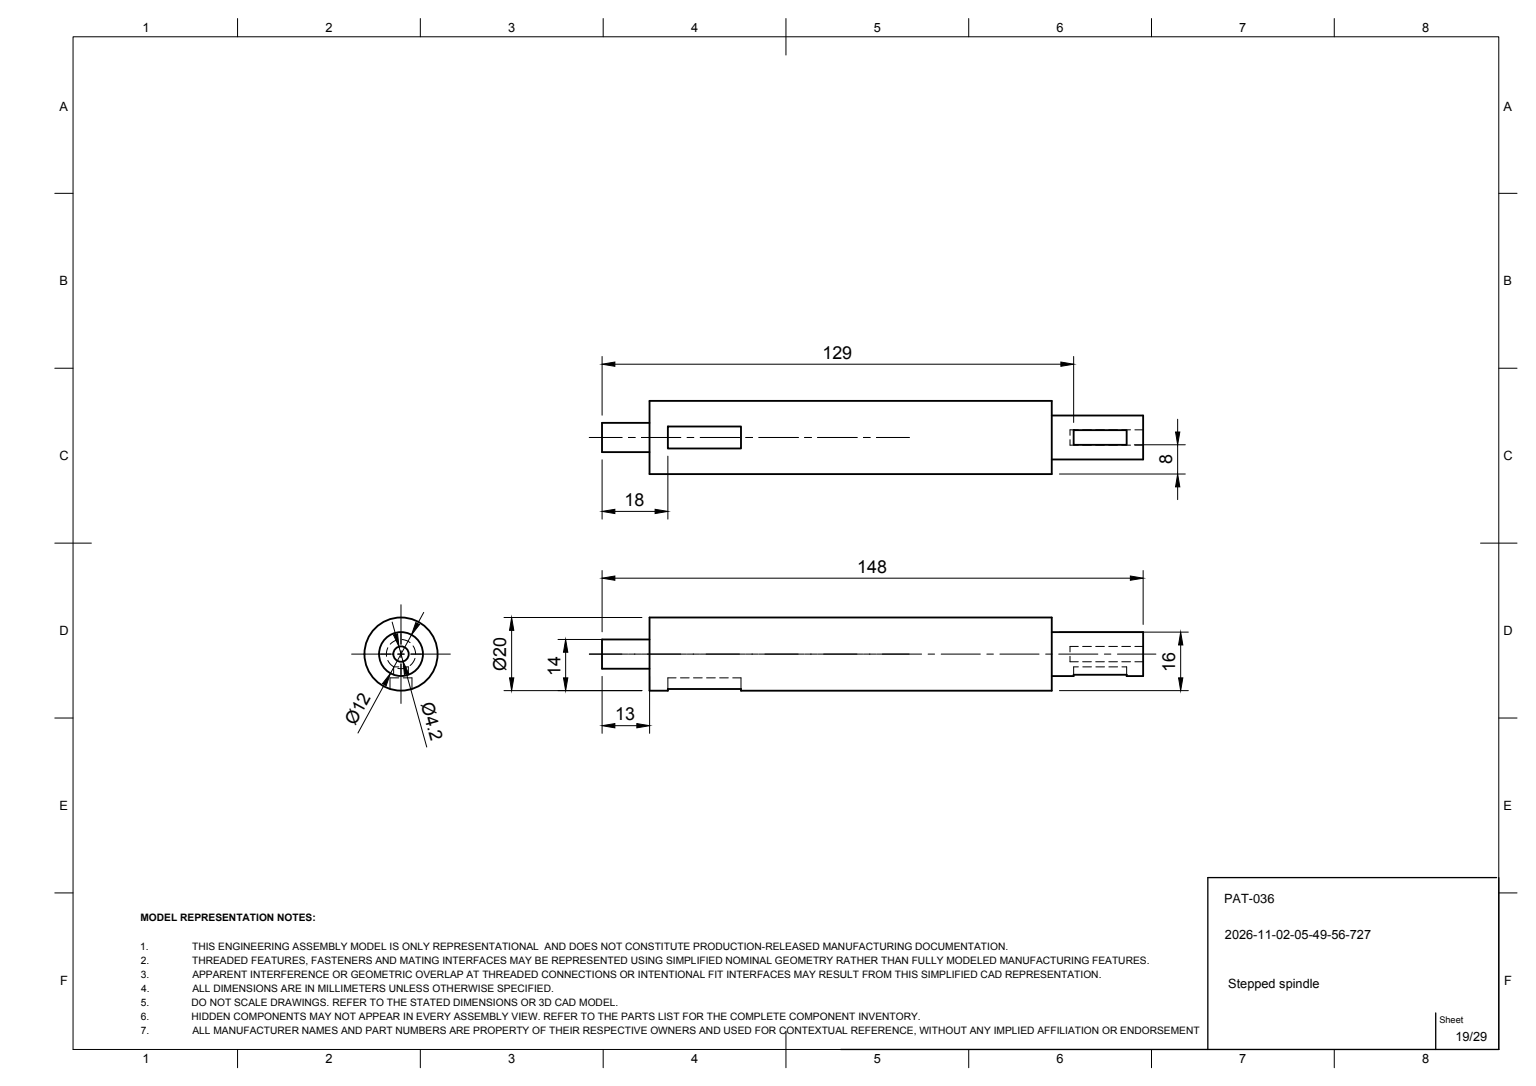
ISO-10303-21;
HEADER;
/* Generated by software containing ST-Developer
 * from STEP Tools, Inc. (www.steptools.com) 
 */

FILE_DESCRIPTION(
/* description */ ('Flange-mounted spindle'),
/* implementation_level */ '2;1');

FILE_NAME(
/* name */ 'Stepped spindle.step',
/* time_stamp */ '2026-10-27T10:49:51-07:00',
/* author */ (''),
/* organization */ (''),
/* preprocessor_version */ 'ST-DEVELOPER v20.2',
/* originating_system */ 'Autodesk Translation Framework v15.17.0.0',
/* authorisation */ '');

FILE_SCHEMA (('AUTOMOTIVE_DESIGN { 1 0 10303 214 3 1 1 }'));
ENDSEC;

DATA;
#10=MECHANICAL_DESIGN_GEOMETRIC_PRESENTATION_REPRESENTATION('',(#351),#11764);
#296=SHAPE_REPRESENTATION_RELATIONSHIP('SRR','None',#11894,#323);
#323=ADVANCED_BREP_SHAPE_REPRESENTATION('',(#377),#11749);
#351=STYLED_ITEM('',(#12085),#377);
#377=MANIFOLD_SOLID_BREP('Body1',#6145);
#452=FACE_BOUND('',#1216,.T.);
#453=FACE_BOUND('',#1218,.T.);
#454=FACE_BOUND('',#1220,.T.);
#455=FACE_BOUND('',#1222,.T.);
#456=FACE_BOUND('',#1224,.T.);
#579=PLANE('',#6676);
#580=PLANE('',#6677);
#581=PLANE('',#6679);
#582=PLANE('',#6680);
#583=PLANE('',#6681);
#584=PLANE('',#6686);
#585=PLANE('',#6687);
#586=PLANE('',#6688);
#587=PLANE('',#6690);
#588=PLANE('',#6691);
#589=PLANE('',#6692);
#590=PLANE('',#6697);
#591=PLANE('',#6701);
#592=PLANE('',#6705);
#593=PLANE('',#6706);
#795=FACE_OUTER_BOUND('',#1201,.T.);
#796=FACE_OUTER_BOUND('',#1202,.T.);
#797=FACE_OUTER_BOUND('',#1203,.T.);
#798=FACE_OUTER_BOUND('',#1204,.T.);
#799=FACE_OUTER_BOUND('',#1205,.T.);
#800=FACE_OUTER_BOUND('',#1206,.T.);
#801=FACE_OUTER_BOUND('',#1207,.T.);
#802=FACE_OUTER_BOUND('',#1208,.T.);
#803=FACE_OUTER_BOUND('',#1209,.T.);
#804=FACE_OUTER_BOUND('',#1210,.T.);
#805=FACE_OUTER_BOUND('',#1211,.T.);
#806=FACE_OUTER_BOUND('',#1212,.T.);
#807=FACE_OUTER_BOUND('',#1213,.T.);
#808=FACE_OUTER_BOUND('',#1214,.T.);
#809=FACE_OUTER_BOUND('',#1215,.T.);
#810=FACE_OUTER_BOUND('',#1217,.T.);
#811=FACE_OUTER_BOUND('',#1219,.T.);
#812=FACE_OUTER_BOUND('',#1221,.T.);
#813=FACE_OUTER_BOUND('',#1223,.T.);
#1201=EDGE_LOOP('',(#4527,#4528,#4529,#4530));
#1202=EDGE_LOOP('',(#4531,#4532,#4533,#4534));
#1203=EDGE_LOOP('',(#4535,#4536,#4537,#4538));
#1204=EDGE_LOOP('',(#4539,#4540,#4541,#4542));
#1205=EDGE_LOOP('',(#4543,#4544,#4545,#4546));
#1206=EDGE_LOOP('',(#4547,#4548,#4549,#4550));
#1207=EDGE_LOOP('',(#4551));
#1208=EDGE_LOOP('',(#4552,#4553,#4554,#4555));
#1209=EDGE_LOOP('',(#4556,#4557,#4558,#4559));
#1210=EDGE_LOOP('',(#4560,#4561,#4562,#4563));
#1211=EDGE_LOOP('',(#4564,#4565,#4566,#4567));
#1212=EDGE_LOOP('',(#4568,#4569,#4570,#4571));
#1213=EDGE_LOOP('',(#4572,#4573,#4574,#4575));
#1214=EDGE_LOOP('',(#4576));
#1215=EDGE_LOOP('',(#4577,#4578,#4579,#4580));
#1216=EDGE_LOOP('',(#4581,#4582,#4583,#4584));
#1217=EDGE_LOOP('',(#4585));
#1218=EDGE_LOOP('',(#4586));
#1219=EDGE_LOOP('',(#4587,#4588,#4589,#4590));
#1220=EDGE_LOOP('',(#4591,#4592,#4593,#4594));
#1221=EDGE_LOOP('',(#4595));
#1222=EDGE_LOOP('',(#4596));
#1223=EDGE_LOOP('',(#4597));
#1224=EDGE_LOOP('',(#4598));
#1639=LINE('',#10119,#2061);
#1640=LINE('',#10121,#2062);
#1641=LINE('',#10123,#2063);
#1642=LINE('',#10124,#2064);
#1643=LINE('',#10129,#2065);
#1644=LINE('',#10130,#2066);
#1645=LINE('',#10133,#2067);
#1646=LINE('',#10135,#2068);
#1647=LINE('',#10136,#2069);
#1648=LINE('',#10138,#2070);
#1649=LINE('',#10145,#2071);
#1650=LINE('',#10151,#2072);
#1651=LINE('',#10153,#2073);
#1652=LINE('',#10155,#2074);
#1653=LINE('',#10156,#2075);
#1654=LINE('',#10161,#2076);
#1655=LINE('',#10162,#2077);
#1656=LINE('',#10165,#2078);
#1657=LINE('',#10167,#2079);
#1658=LINE('',#10168,#2080);
#1659=LINE('',#10170,#2081);
#1660=LINE('',#10177,#2082);
#1661=LINE('',#10184,#2083);
#1662=LINE('',#10191,#2084);
#2061=VECTOR('',#7804,1.);
#2062=VECTOR('',#7805,1.);
#2063=VECTOR('',#7806,1.);
#2064=VECTOR('',#7807,1.);
#2065=VECTOR('',#7812,1.);
#2066=VECTOR('',#7813,1.);
#2067=VECTOR('',#7816,1.);
#2068=VECTOR('',#7817,1.);
#2069=VECTOR('',#7818,1.);
#2070=VECTOR('',#7821,1.);
#2071=VECTOR('',#7830,0.21);
#2072=VECTOR('',#7837,1.);
#2073=VECTOR('',#7838,1.);
#2074=VECTOR('',#7839,1.);
#2075=VECTOR('',#7840,1.);
#2076=VECTOR('',#7845,1.);
#2077=VECTOR('',#7846,1.);
#2078=VECTOR('',#7849,1.);
#2079=VECTOR('',#7850,1.);
#2080=VECTOR('',#7851,1.);
#2081=VECTOR('',#7854,1.);
#2082=VECTOR('',#7863,0.4);
#2083=VECTOR('',#7872,0.6);
#2084=VECTOR('',#7881,1.);
#2400=CIRCLE('',#6678,1.);
#2401=CIRCLE('',#6682,1.);
#2402=CIRCLE('',#6684,0.21);
#2403=CIRCLE('',#6685,0.21);
#2404=CIRCLE('',#6689,0.6);
#2405=CIRCLE('',#6693,0.6);
#2406=CIRCLE('',#6695,0.4);
#2407=CIRCLE('',#6696,0.4);
#2408=CIRCLE('',#6699,0.6);
#2409=CIRCLE('',#6700,0.6);
#2410=CIRCLE('',#6703,1.);
#2411=CIRCLE('',#6704,1.);
#2828=VERTEX_POINT('',#10117);
#2829=VERTEX_POINT('',#10118);
#2830=VERTEX_POINT('',#10120);
#2831=VERTEX_POINT('',#10122);
#2832=VERTEX_POINT('',#10126);
#2833=VERTEX_POINT('',#10128);
#2834=VERTEX_POINT('',#10132);
#2835=VERTEX_POINT('',#10134);
#2836=VERTEX_POINT('',#10142);
#2837=VERTEX_POINT('',#10144);
#2838=VERTEX_POINT('',#10149);
#2839=VERTEX_POINT('',#10150);
#2840=VERTEX_POINT('',#10152);
#2841=VERTEX_POINT('',#10154);
#2842=VERTEX_POINT('',#10158);
#2843=VERTEX_POINT('',#10160);
#2844=VERTEX_POINT('',#10164);
#2845=VERTEX_POINT('',#10166);
#2846=VERTEX_POINT('',#10174);
#2847=VERTEX_POINT('',#10176);
#2848=VERTEX_POINT('',#10181);
#2849=VERTEX_POINT('',#10183);
#2850=VERTEX_POINT('',#10188);
#2851=VERTEX_POINT('',#10190);
#3456=EDGE_CURVE('',#2828,#2829,#1639,.T.);
#3457=EDGE_CURVE('',#2828,#2830,#1640,.T.);
#3458=EDGE_CURVE('',#2831,#2830,#1641,.T.);
#3459=EDGE_CURVE('',#2831,#2829,#1642,.T.);
#3460=EDGE_CURVE('',#2829,#2832,#2400,.T.);
#3461=EDGE_CURVE('',#2833,#2831,#1643,.T.);
#3462=EDGE_CURVE('',#2832,#2833,#1644,.T.);
#3463=EDGE_CURVE('',#2832,#2834,#1645,.T.);
#3464=EDGE_CURVE('',#2833,#2835,#1646,.T.);
#3465=EDGE_CURVE('',#2835,#2834,#1647,.T.);
#3466=EDGE_CURVE('',#2830,#2835,#1648,.T.);
#3467=EDGE_CURVE('',#2834,#2828,#2401,.T.);
#3468=EDGE_CURVE('',#2836,#2836,#2402,.T.);
#3469=EDGE_CURVE('',#2836,#2837,#1649,.T.);
#3470=EDGE_CURVE('',#2837,#2837,#2403,.T.);
#3471=EDGE_CURVE('',#2838,#2839,#1650,.T.);
#3472=EDGE_CURVE('',#2838,#2840,#1651,.T.);
#3473=EDGE_CURVE('',#2841,#2840,#1652,.T.);
#3474=EDGE_CURVE('',#2841,#2839,#1653,.T.);
#3475=EDGE_CURVE('',#2839,#2842,#2404,.T.);
#3476=EDGE_CURVE('',#2843,#2841,#1654,.T.);
#3477=EDGE_CURVE('',#2842,#2843,#1655,.T.);
#3478=EDGE_CURVE('',#2842,#2844,#1656,.T.);
#3479=EDGE_CURVE('',#2843,#2845,#1657,.T.);
#3480=EDGE_CURVE('',#2845,#2844,#1658,.T.);
#3481=EDGE_CURVE('',#2840,#2845,#1659,.T.);
#3482=EDGE_CURVE('',#2844,#2838,#2405,.T.);
#3483=EDGE_CURVE('',#2846,#2846,#2406,.T.);
#3484=EDGE_CURVE('',#2846,#2847,#1660,.T.);
#3485=EDGE_CURVE('',#2847,#2847,#2407,.T.);
#3486=EDGE_CURVE('',#2848,#2848,#2408,.T.);
#3487=EDGE_CURVE('',#2848,#2849,#1661,.T.);
#3488=EDGE_CURVE('',#2849,#2849,#2409,.T.);
#3489=EDGE_CURVE('',#2850,#2850,#2410,.T.);
#3490=EDGE_CURVE('',#2850,#2851,#1662,.T.);
#3491=EDGE_CURVE('',#2851,#2851,#2411,.T.);
#4527=ORIENTED_EDGE('',*,*,#3456,.F.);
#4528=ORIENTED_EDGE('',*,*,#3457,.T.);
#4529=ORIENTED_EDGE('',*,*,#3458,.F.);
#4530=ORIENTED_EDGE('',*,*,#3459,.T.);
#4531=ORIENTED_EDGE('',*,*,#3460,.F.);
#4532=ORIENTED_EDGE('',*,*,#3459,.F.);
#4533=ORIENTED_EDGE('',*,*,#3461,.F.);
#4534=ORIENTED_EDGE('',*,*,#3462,.F.);
#4535=ORIENTED_EDGE('',*,*,#3463,.F.);
#4536=ORIENTED_EDGE('',*,*,#3462,.T.);
#4537=ORIENTED_EDGE('',*,*,#3464,.T.);
#4538=ORIENTED_EDGE('',*,*,#3465,.T.);
#4539=ORIENTED_EDGE('',*,*,#3461,.T.);
#4540=ORIENTED_EDGE('',*,*,#3458,.T.);
#4541=ORIENTED_EDGE('',*,*,#3466,.T.);
#4542=ORIENTED_EDGE('',*,*,#3464,.F.);
#4543=ORIENTED_EDGE('',*,*,#3467,.F.);
#4544=ORIENTED_EDGE('',*,*,#3465,.F.);
#4545=ORIENTED_EDGE('',*,*,#3466,.F.);
#4546=ORIENTED_EDGE('',*,*,#3457,.F.);
#4547=ORIENTED_EDGE('',*,*,#3468,.F.);
#4548=ORIENTED_EDGE('',*,*,#3469,.T.);
#4549=ORIENTED_EDGE('',*,*,#3470,.T.);
#4550=ORIENTED_EDGE('',*,*,#3469,.F.);
#4551=ORIENTED_EDGE('',*,*,#3470,.F.);
#4552=ORIENTED_EDGE('',*,*,#3471,.F.);
#4553=ORIENTED_EDGE('',*,*,#3472,.T.);
#4554=ORIENTED_EDGE('',*,*,#3473,.F.);
#4555=ORIENTED_EDGE('',*,*,#3474,.T.);
#4556=ORIENTED_EDGE('',*,*,#3475,.F.);
#4557=ORIENTED_EDGE('',*,*,#3474,.F.);
#4558=ORIENTED_EDGE('',*,*,#3476,.F.);
#4559=ORIENTED_EDGE('',*,*,#3477,.F.);
#4560=ORIENTED_EDGE('',*,*,#3478,.F.);
#4561=ORIENTED_EDGE('',*,*,#3477,.T.);
#4562=ORIENTED_EDGE('',*,*,#3479,.T.);
#4563=ORIENTED_EDGE('',*,*,#3480,.T.);
#4564=ORIENTED_EDGE('',*,*,#3476,.T.);
#4565=ORIENTED_EDGE('',*,*,#3473,.T.);
#4566=ORIENTED_EDGE('',*,*,#3481,.T.);
#4567=ORIENTED_EDGE('',*,*,#3479,.F.);
#4568=ORIENTED_EDGE('',*,*,#3482,.F.);
#4569=ORIENTED_EDGE('',*,*,#3480,.F.);
#4570=ORIENTED_EDGE('',*,*,#3481,.F.);
#4571=ORIENTED_EDGE('',*,*,#3472,.F.);
#4572=ORIENTED_EDGE('',*,*,#3483,.F.);
#4573=ORIENTED_EDGE('',*,*,#3484,.T.);
#4574=ORIENTED_EDGE('',*,*,#3485,.F.);
#4575=ORIENTED_EDGE('',*,*,#3484,.F.);
#4576=ORIENTED_EDGE('',*,*,#3483,.T.);
#4577=ORIENTED_EDGE('',*,*,#3486,.F.);
#4578=ORIENTED_EDGE('',*,*,#3487,.T.);
#4579=ORIENTED_EDGE('',*,*,#3488,.T.);
#4580=ORIENTED_EDGE('',*,*,#3487,.F.);
#4581=ORIENTED_EDGE('',*,*,#3478,.T.);
#4582=ORIENTED_EDGE('',*,*,#3482,.T.);
#4583=ORIENTED_EDGE('',*,*,#3471,.T.);
#4584=ORIENTED_EDGE('',*,*,#3475,.T.);
#4585=ORIENTED_EDGE('',*,*,#3488,.F.);
#4586=ORIENTED_EDGE('',*,*,#3468,.T.);
#4587=ORIENTED_EDGE('',*,*,#3489,.F.);
#4588=ORIENTED_EDGE('',*,*,#3490,.T.);
#4589=ORIENTED_EDGE('',*,*,#3491,.T.);
#4590=ORIENTED_EDGE('',*,*,#3490,.F.);
#4591=ORIENTED_EDGE('',*,*,#3463,.T.);
#4592=ORIENTED_EDGE('',*,*,#3467,.T.);
#4593=ORIENTED_EDGE('',*,*,#3456,.T.);
#4594=ORIENTED_EDGE('',*,*,#3460,.T.);
#4595=ORIENTED_EDGE('',*,*,#3489,.T.);
#4596=ORIENTED_EDGE('',*,*,#3485,.T.);
#4597=ORIENTED_EDGE('',*,*,#3491,.F.);
#4598=ORIENTED_EDGE('',*,*,#3486,.T.);
#5664=CYLINDRICAL_SURFACE('',#6683,0.21);
#5665=CYLINDRICAL_SURFACE('',#6694,0.4);
#5666=CYLINDRICAL_SURFACE('',#6698,0.6);
#5667=CYLINDRICAL_SURFACE('',#6702,1.);
#5906=ADVANCED_FACE('',(#795),#579,.F.);
#5907=ADVANCED_FACE('',(#796),#580,.T.);
#5908=ADVANCED_FACE('',(#797),#581,.F.);
#5909=ADVANCED_FACE('',(#798),#582,.F.);
#5910=ADVANCED_FACE('',(#799),#583,.F.);
#5911=ADVANCED_FACE('',(#800),#5664,.F.);
#5912=ADVANCED_FACE('',(#801),#584,.F.);
#5913=ADVANCED_FACE('',(#802),#585,.F.);
#5914=ADVANCED_FACE('',(#803),#586,.T.);
#5915=ADVANCED_FACE('',(#804),#587,.F.);
#5916=ADVANCED_FACE('',(#805),#588,.F.);
#5917=ADVANCED_FACE('',(#806),#589,.F.);
#5918=ADVANCED_FACE('',(#807),#5665,.T.);
#5919=ADVANCED_FACE('',(#808),#590,.T.);
#5920=ADVANCED_FACE('',(#809,#452),#5666,.T.);
#5921=ADVANCED_FACE('',(#810,#453),#591,.F.);
#5922=ADVANCED_FACE('',(#811,#454),#5667,.T.);
#5923=ADVANCED_FACE('',(#812,#455),#592,.T.);
#5924=ADVANCED_FACE('',(#813,#456),#593,.F.);
#6145=CLOSED_SHELL('',(#5906,#5907,#5908,#5909,#5910,#5911,#5912,#5913,
#5914,#5915,#5916,#5917,#5918,#5919,#5920,#5921,#5922,#5923,#5924));
#6675=AXIS2_PLACEMENT_3D('',#10115,#7800,#7801);
#6676=AXIS2_PLACEMENT_3D('',#10116,#7802,#7803);
#6677=AXIS2_PLACEMENT_3D('',#10125,#7808,#7809);
#6678=AXIS2_PLACEMENT_3D('',#10127,#7810,#7811);
#6679=AXIS2_PLACEMENT_3D('',#10131,#7814,#7815);
#6680=AXIS2_PLACEMENT_3D('',#10137,#7819,#7820);
#6681=AXIS2_PLACEMENT_3D('',#10139,#7822,#7823);
#6682=AXIS2_PLACEMENT_3D('',#10140,#7824,#7825);
#6683=AXIS2_PLACEMENT_3D('',#10141,#7826,#7827);
#6684=AXIS2_PLACEMENT_3D('',#10143,#7828,#7829);
#6685=AXIS2_PLACEMENT_3D('',#10146,#7831,#7832);
#6686=AXIS2_PLACEMENT_3D('',#10147,#7833,#7834);
#6687=AXIS2_PLACEMENT_3D('',#10148,#7835,#7836);
#6688=AXIS2_PLACEMENT_3D('',#10157,#7841,#7842);
#6689=AXIS2_PLACEMENT_3D('',#10159,#7843,#7844);
#6690=AXIS2_PLACEMENT_3D('',#10163,#7847,#7848);
#6691=AXIS2_PLACEMENT_3D('',#10169,#7852,#7853);
#6692=AXIS2_PLACEMENT_3D('',#10171,#7855,#7856);
#6693=AXIS2_PLACEMENT_3D('',#10172,#7857,#7858);
#6694=AXIS2_PLACEMENT_3D('',#10173,#7859,#7860);
#6695=AXIS2_PLACEMENT_3D('',#10175,#7861,#7862);
#6696=AXIS2_PLACEMENT_3D('',#10178,#7864,#7865);
#6697=AXIS2_PLACEMENT_3D('',#10179,#7866,#7867);
#6698=AXIS2_PLACEMENT_3D('',#10180,#7868,#7869);
#6699=AXIS2_PLACEMENT_3D('',#10182,#7870,#7871);
#6700=AXIS2_PLACEMENT_3D('',#10185,#7873,#7874);
#6701=AXIS2_PLACEMENT_3D('',#10186,#7875,#7876);
#6702=AXIS2_PLACEMENT_3D('',#10187,#7877,#7878);
#6703=AXIS2_PLACEMENT_3D('',#10189,#7879,#7880);
#6704=AXIS2_PLACEMENT_3D('',#10192,#7882,#7883);
#6705=AXIS2_PLACEMENT_3D('',#10193,#7884,#7885);
#6706=AXIS2_PLACEMENT_3D('',#10194,#7886,#7887);
#7800=DIRECTION('axis',(0.,0.,1.));
#7801=DIRECTION('refdir',(1.,0.,0.));
#7802=DIRECTION('center_axis',(-1.,0.,0.));
#7803=DIRECTION('ref_axis',(0.,0.,1.));
#7804=DIRECTION('',(0.,-1.,0.));
#7805=DIRECTION('',(0.,0.,1.));
#7806=DIRECTION('',(0.,1.,0.));
#7807=DIRECTION('',(0.,0.,-1.));
#7808=DIRECTION('center_axis',(0.,1.,0.));
#7809=DIRECTION('ref_axis',(1.,0.,0.));
#7810=DIRECTION('center_axis',(0.,-1.,0.));
#7811=DIRECTION('ref_axis',(1.,0.,0.));
#7812=DIRECTION('',(-1.,0.,0.));
#7813=DIRECTION('',(0.,0.,1.));
#7814=DIRECTION('center_axis',(1.,0.,0.));
#7815=DIRECTION('ref_axis',(0.,0.,-1.));
#7816=DIRECTION('',(0.,1.,0.));
#7817=DIRECTION('',(0.,1.,0.));
#7818=DIRECTION('',(0.,0.,-1.));
#7819=DIRECTION('center_axis',(0.,0.,1.));
#7820=DIRECTION('ref_axis',(1.,0.,0.));
#7821=DIRECTION('',(1.,0.,0.));
#7822=DIRECTION('center_axis',(0.,1.,0.));
#7823=DIRECTION('ref_axis',(0.,0.,1.));
#7824=DIRECTION('center_axis',(0.,1.,0.));
#7825=DIRECTION('ref_axis',(1.,0.,0.));
#7826=DIRECTION('center_axis',(0.,1.,0.));
#7827=DIRECTION('ref_axis',(1.,0.,0.));
#7828=DIRECTION('center_axis',(0.,1.,0.));
#7829=DIRECTION('ref_axis',(1.,0.,0.));
#7830=DIRECTION('',(0.,1.,0.));
#7831=DIRECTION('center_axis',(0.,1.,0.));
#7832=DIRECTION('ref_axis',(1.,0.,0.));
#7833=DIRECTION('center_axis',(0.,1.,0.));
#7834=DIRECTION('ref_axis',(1.,0.,0.));
#7835=DIRECTION('center_axis',(-1.,0.,0.));
#7836=DIRECTION('ref_axis',(0.,0.,1.));
#7837=DIRECTION('',(0.,-1.,0.));
#7838=DIRECTION('',(0.,0.,1.));
#7839=DIRECTION('',(0.,1.,0.));
#7840=DIRECTION('',(0.,0.,-1.));
#7841=DIRECTION('center_axis',(0.,1.,0.));
#7842=DIRECTION('ref_axis',(1.,0.,0.));
#7843=DIRECTION('center_axis',(0.,-1.,0.));
#7844=DIRECTION('ref_axis',(1.,0.,0.));
#7845=DIRECTION('',(-1.,0.,0.));
#7846=DIRECTION('',(0.,0.,1.));
#7847=DIRECTION('center_axis',(1.,0.,0.));
#7848=DIRECTION('ref_axis',(0.,0.,-1.));
#7849=DIRECTION('',(0.,1.,0.));
#7850=DIRECTION('',(0.,1.,0.));
#7851=DIRECTION('',(0.,0.,-1.));
#7852=DIRECTION('center_axis',(0.,0.,1.));
#7853=DIRECTION('ref_axis',(1.,0.,0.));
#7854=DIRECTION('',(1.,0.,0.));
#7855=DIRECTION('center_axis',(0.,1.,0.));
#7856=DIRECTION('ref_axis',(0.,0.,1.));
#7857=DIRECTION('center_axis',(0.,1.,0.));
#7858=DIRECTION('ref_axis',(1.,0.,0.));
#7859=DIRECTION('center_axis',(0.,1.,0.));
#7860=DIRECTION('ref_axis',(1.,0.,0.));
#7861=DIRECTION('center_axis',(0.,1.,0.));
#7862=DIRECTION('ref_axis',(1.,0.,0.));
#7863=DIRECTION('',(0.,-1.,0.));
#7864=DIRECTION('center_axis',(0.,-1.,0.));
#7865=DIRECTION('ref_axis',(1.,0.,0.));
#7866=DIRECTION('center_axis',(0.,1.,0.));
#7867=DIRECTION('ref_axis',(1.,0.,0.));
#7868=DIRECTION('center_axis',(0.,1.,0.));
#7869=DIRECTION('ref_axis',(1.,0.,0.));
#7870=DIRECTION('center_axis',(0.,1.,0.));
#7871=DIRECTION('ref_axis',(1.,0.,0.));
#7872=DIRECTION('',(0.,-1.,0.));
#7873=DIRECTION('center_axis',(0.,1.,0.));
#7874=DIRECTION('ref_axis',(1.,0.,0.));
#7875=DIRECTION('center_axis',(0.,1.,0.));
#7876=DIRECTION('ref_axis',(1.,0.,0.));
#7877=DIRECTION('center_axis',(0.,1.,0.));
#7878=DIRECTION('ref_axis',(1.,0.,0.));
#7879=DIRECTION('center_axis',(0.,1.,0.));
#7880=DIRECTION('ref_axis',(1.,0.,0.));
#7881=DIRECTION('',(0.,-1.,0.));
#7882=DIRECTION('center_axis',(0.,1.,0.));
#7883=DIRECTION('ref_axis',(1.,0.,0.));
#7884=DIRECTION('center_axis',(0.,1.,0.));
#7885=DIRECTION('ref_axis',(1.,0.,0.));
#7886=DIRECTION('center_axis',(0.,1.,0.));
#7887=DIRECTION('ref_axis',(1.,0.,0.));
#10115=CARTESIAN_POINT('',(0.,0.,0.));
#10116=CARTESIAN_POINT('Origin',(-0.3,4.,6.9));
#10117=CARTESIAN_POINT('',(-0.3,6.,7.04606079858305));
#10118=CARTESIAN_POINT('',(-0.3,4.,7.04606079858305));
#10119=CARTESIAN_POINT('',(-0.3,-4.5,7.04606079858305));
#10120=CARTESIAN_POINT('',(-0.3,6.,7.35));
#10121=CARTESIAN_POINT('',(-0.3,6.,7.35));
#10122=CARTESIAN_POINT('',(-0.3,4.,7.35));
#10123=CARTESIAN_POINT('',(-0.3,4.,7.35));
#10124=CARTESIAN_POINT('',(-0.3,4.,7.35));
#10125=CARTESIAN_POINT('Origin',(0.,4.,7.125));
#10126=CARTESIAN_POINT('',(0.3,4.,7.04606079858305));
#10127=CARTESIAN_POINT('Origin',(0.,4.,8.));
#10128=CARTESIAN_POINT('',(0.3,4.,7.35));
#10129=CARTESIAN_POINT('',(0.3,4.,7.35));
#10130=CARTESIAN_POINT('',(0.3,4.,6.9));
#10131=CARTESIAN_POINT('Origin',(0.3,4.,7.35));
#10132=CARTESIAN_POINT('',(0.3,6.,7.04606079858305));
#10133=CARTESIAN_POINT('',(0.3,-4.5,7.04606079858305));
#10134=CARTESIAN_POINT('',(0.3,6.,7.35));
#10135=CARTESIAN_POINT('',(0.3,4.,7.35));
#10136=CARTESIAN_POINT('',(0.3,6.,6.9));
#10137=CARTESIAN_POINT('Origin',(-0.3,4.,7.35));
#10138=CARTESIAN_POINT('',(0.3,6.,7.35));
#10139=CARTESIAN_POINT('Origin',(0.,6.,7.125));
#10140=CARTESIAN_POINT('Origin',(0.,6.,8.));
#10141=CARTESIAN_POINT('Origin',(0.,-7.1,8.));
#10142=CARTESIAN_POINT('',(-0.21,-7.,8.));
#10143=CARTESIAN_POINT('Origin',(0.,-7.,8.));
#10144=CARTESIAN_POINT('',(-0.21,-5.,8.));
#10145=CARTESIAN_POINT('',(-0.21,-7.1,8.));
#10146=CARTESIAN_POINT('Origin',(0.,-5.,8.));
#10147=CARTESIAN_POINT('Origin',(0.,-5.,8.));
#10148=CARTESIAN_POINT('Origin',(-0.2,-6.55,7.3));
#10149=CARTESIAN_POINT('',(-0.2,-5.1,7.43431457505076));
#10150=CARTESIAN_POINT('',(-0.2,-6.55,7.43431457505076));
#10151=CARTESIAN_POINT('',(-0.2,-7.,7.43431457505076));
#10152=CARTESIAN_POINT('',(-0.2,-5.1,7.65));
#10153=CARTESIAN_POINT('',(-0.2,-5.1,7.65));
#10154=CARTESIAN_POINT('',(-0.2,-6.55,7.65));
#10155=CARTESIAN_POINT('',(-0.2,-6.55,7.65));
#10156=CARTESIAN_POINT('',(-0.2,-6.55,7.65));
#10157=CARTESIAN_POINT('Origin',(0.,-6.55,7.475));
#10158=CARTESIAN_POINT('',(0.2,-6.55,7.43431457505076));
#10159=CARTESIAN_POINT('Origin',(0.,-6.55,8.));
#10160=CARTESIAN_POINT('',(0.2,-6.55,7.65));
#10161=CARTESIAN_POINT('',(0.2,-6.55,7.65));
#10162=CARTESIAN_POINT('',(0.2,-6.55,7.3));
#10163=CARTESIAN_POINT('Origin',(0.2,-6.55,7.65));
#10164=CARTESIAN_POINT('',(0.2,-5.1,7.43431457505076));
#10165=CARTESIAN_POINT('',(0.2,-7.,7.43431457505076));
#10166=CARTESIAN_POINT('',(0.2,-5.1,7.65));
#10167=CARTESIAN_POINT('',(0.2,-6.55,7.65));
#10168=CARTESIAN_POINT('',(0.2,-5.1,7.3));
#10169=CARTESIAN_POINT('Origin',(-0.2,-6.55,7.65));
#10170=CARTESIAN_POINT('',(0.2,-5.1,7.65));
#10171=CARTESIAN_POINT('Origin',(0.,-5.1,7.475));
#10172=CARTESIAN_POINT('Origin',(0.,-5.1,8.));
#10173=CARTESIAN_POINT('Origin',(0.,6.5,8.));
#10174=CARTESIAN_POINT('',(-0.4,7.8,8.));
#10175=CARTESIAN_POINT('Origin',(0.,7.8,8.));
#10176=CARTESIAN_POINT('',(-0.4,6.5,8.));
#10177=CARTESIAN_POINT('',(-0.4,6.5,8.));
#10178=CARTESIAN_POINT('Origin',(0.,6.5,8.));
#10179=CARTESIAN_POINT('Origin',(0.,7.8,8.));
#10180=CARTESIAN_POINT('Origin',(0.,-7.,8.));
#10181=CARTESIAN_POINT('',(-0.6,-4.5,8.));
#10182=CARTESIAN_POINT('Origin',(0.,-4.5,8.));
#10183=CARTESIAN_POINT('',(-0.6,-7.,8.));
#10184=CARTESIAN_POINT('',(-0.6,-7.,8.));
#10185=CARTESIAN_POINT('Origin',(0.,-7.,8.));
#10186=CARTESIAN_POINT('Origin',(0.,-7.,8.));
#10187=CARTESIAN_POINT('Origin',(0.,-4.5,8.));
#10188=CARTESIAN_POINT('',(-1.,6.5,8.));
#10189=CARTESIAN_POINT('Origin',(0.,6.5,8.));
#10190=CARTESIAN_POINT('',(-1.,-4.5,8.));
#10191=CARTESIAN_POINT('',(-1.,-4.5,8.));
#10192=CARTESIAN_POINT('Origin',(0.,-4.5,8.));
#10193=CARTESIAN_POINT('Origin',(0.,6.5,8.));
#10194=CARTESIAN_POINT('Origin',(0.,-4.5,8.));
#11717=UNCERTAINTY_MEASURE_WITH_UNIT(LENGTH_MEASURE(0.001),#11765,
'DISTANCE_ACCURACY_VALUE',
'Maximum model space distance between geometric entities at asserted c
onnectivities');
#11732=UNCERTAINTY_MEASURE_WITH_UNIT(LENGTH_MEASURE(0.001),#11765,
'DISTANCE_ACCURACY_VALUE',
'Maximum model space distance between geometric entities at asserted c
onnectivities');
#11749=(
GEOMETRIC_REPRESENTATION_CONTEXT(3)
GLOBAL_UNCERTAINTY_ASSIGNED_CONTEXT((#11717))
GLOBAL_UNIT_ASSIGNED_CONTEXT((#11765,#11767,#11768))
REPRESENTATION_CONTEXT('','3D')
);
#11764=(
GEOMETRIC_REPRESENTATION_CONTEXT(3)
GLOBAL_UNCERTAINTY_ASSIGNED_CONTEXT((#11732))
GLOBAL_UNIT_ASSIGNED_CONTEXT((#11765,#11767,#11768))
REPRESENTATION_CONTEXT('','3D')
);
#11765=(
LENGTH_UNIT()
NAMED_UNIT(*)
SI_UNIT(.CENTI.,.METRE.)
);
#11767=(
NAMED_UNIT(*)
PLANE_ANGLE_UNIT()
SI_UNIT($,.RADIAN.)
);
#11768=(
NAMED_UNIT(*)
SI_UNIT($,.STERADIAN.)
SOLID_ANGLE_UNIT()
);
#11785=SHAPE_DEFINITION_REPRESENTATION(#11818,#11894);
#11818=PRODUCT_DEFINITION_SHAPE('',$,#11926);
#11894=SHAPE_REPRESENTATION('',(#6675),#11749);
#11909=PRODUCT_DEFINITION_CONTEXT('part definition',#12004,'design');
#11926=PRODUCT_DEFINITION('Stepped spindle','Stepped spindle',#11957,
#11909);
#11957=PRODUCT_DEFINITION_FORMATION('',$,#12022);
#12004=APPLICATION_CONTEXT(
'Core Data for Automotive Mechanical Design Process');
#12005=PRODUCT_CONTEXT('part definition',#12004,'mechanical');
#12022=PRODUCT('Stepped spindle','Stepped spindle','Stepped spindle',
(#12005));
#12079=COLOUR_RGB('Light Blue',0.38,0.62,0.78);
#12080=FILL_AREA_STYLE_COLOUR('',#12079);
#12081=FILL_AREA_STYLE('',(#12080));
#12082=SURFACE_STYLE_FILL_AREA(#12081);
#12083=SURFACE_SIDE_STYLE('',(#12082));
#12084=SURFACE_STYLE_USAGE(.BOTH.,#12083);
#12085=PRESENTATION_STYLE_ASSIGNMENT((#12084));
ENDSEC;
END-ISO-10303-21;
